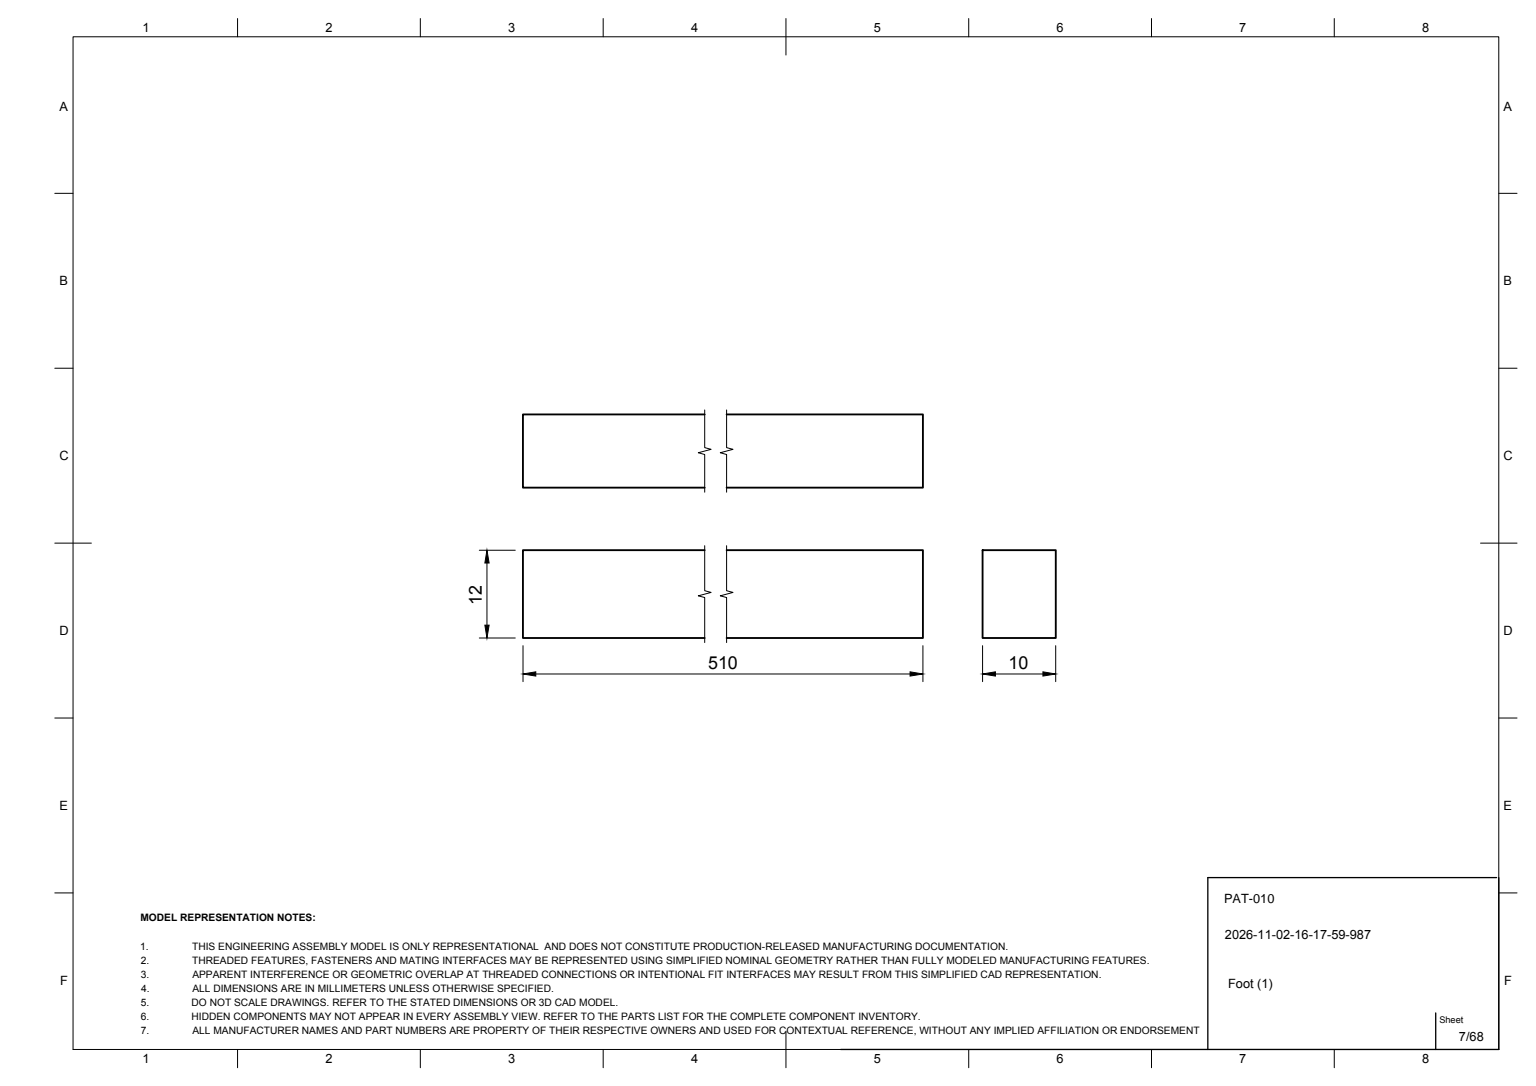
ISO-10303-21;
HEADER;
/* Generated by software containing ST-Developer
 * from STEP Tools, Inc. (www.steptools.com) 
 */

FILE_DESCRIPTION(
/* description */ ('Belt conveyor head drive unit'),
/* implementation_level */ '2;1');

FILE_NAME(
/* name */ 'Foot (1).step',
/* time_stamp */ '2026-10-28T03:26:19-07:00',
/* author */ (''),
/* organization */ (''),
/* preprocessor_version */ 'ST-DEVELOPER v20.2',
/* originating_system */ 'Autodesk Translation Framework v15.17.0.0',
/* authorisation */ '');

FILE_SCHEMA (('AUTOMOTIVE_DESIGN { 1 0 10303 214 3 1 1 }'));
ENDSEC;

DATA;
#10=MECHANICAL_DESIGN_GEOMETRIC_PRESENTATION_REPRESENTATION('',(#849),#27069);
#711=SHAPE_REPRESENTATION_RELATIONSHIP('SRR','None',#27355,#780);
#780=ADVANCED_BREP_SHAPE_REPRESENTATION('',(#934),#26997);
#849=STYLED_ITEM('',(#27811),#934);
#934=MANIFOLD_SOLID_BREP('Body1',#13714);
#1311=PLANE('',#14671);
#1312=PLANE('',#14672);
#1313=PLANE('',#14673);
#1314=PLANE('',#14674);
#1315=PLANE('',#14675);
#1316=PLANE('',#14676);
#1689=FACE_OUTER_BOUND('',#2509,.T.);
#1690=FACE_OUTER_BOUND('',#2510,.T.);
#1691=FACE_OUTER_BOUND('',#2511,.T.);
#1692=FACE_OUTER_BOUND('',#2512,.T.);
#1693=FACE_OUTER_BOUND('',#2513,.T.);
#1694=FACE_OUTER_BOUND('',#2514,.T.);
#2509=EDGE_LOOP('',(#9198,#9199,#9200,#9201));
#2510=EDGE_LOOP('',(#9202,#9203,#9204,#9205));
#2511=EDGE_LOOP('',(#9206,#9207,#9208,#9209));
#2512=EDGE_LOOP('',(#9210,#9211,#9212,#9213));
#2513=EDGE_LOOP('',(#9214,#9215,#9216,#9217));
#2514=EDGE_LOOP('',(#9218,#9219,#9220,#9221));
#3570=LINE('',#21234,#4362);
#3571=LINE('',#21236,#4363);
#3572=LINE('',#21238,#4364);
#3573=LINE('',#21239,#4365);
#3574=LINE('',#21242,#4366);
#3575=LINE('',#21244,#4367);
#3576=LINE('',#21245,#4368);
#3577=LINE('',#21248,#4369);
#3578=LINE('',#21250,#4370);
#3579=LINE('',#21251,#4371);
#3580=LINE('',#21253,#4372);
#3581=LINE('',#21254,#4373);
#4362=VECTOR('',#16726,1.);
#4363=VECTOR('',#16727,1.);
#4364=VECTOR('',#16728,1.);
#4365=VECTOR('',#16729,1.);
#4366=VECTOR('',#16732,1.);
#4367=VECTOR('',#16733,1.);
#4368=VECTOR('',#16734,1.);
#4369=VECTOR('',#16737,1.);
#4370=VECTOR('',#16738,1.);
#4371=VECTOR('',#16739,1.);
#4372=VECTOR('',#16742,1.);
#4373=VECTOR('',#16743,1.);
#6033=VERTEX_POINT('',#21232);
#6034=VERTEX_POINT('',#21233);
#6035=VERTEX_POINT('',#21235);
#6036=VERTEX_POINT('',#21237);
#6037=VERTEX_POINT('',#21241);
#6038=VERTEX_POINT('',#21243);
#6039=VERTEX_POINT('',#21247);
#6040=VERTEX_POINT('',#21249);
#7291=EDGE_CURVE('',#6033,#6034,#3570,.T.);
#7292=EDGE_CURVE('',#6034,#6035,#3571,.T.);
#7293=EDGE_CURVE('',#6036,#6035,#3572,.T.);
#7294=EDGE_CURVE('',#6033,#6036,#3573,.T.);
#7295=EDGE_CURVE('',#6037,#6033,#3574,.T.);
#7296=EDGE_CURVE('',#6038,#6036,#3575,.T.);
#7297=EDGE_CURVE('',#6037,#6038,#3576,.T.);
#7298=EDGE_CURVE('',#6039,#6037,#3577,.T.);
#7299=EDGE_CURVE('',#6040,#6038,#3578,.T.);
#7300=EDGE_CURVE('',#6039,#6040,#3579,.T.);
#7301=EDGE_CURVE('',#6034,#6039,#3580,.T.);
#7302=EDGE_CURVE('',#6035,#6040,#3581,.T.);
#9198=ORIENTED_EDGE('',*,*,#7291,.T.);
#9199=ORIENTED_EDGE('',*,*,#7292,.T.);
#9200=ORIENTED_EDGE('',*,*,#7293,.F.);
#9201=ORIENTED_EDGE('',*,*,#7294,.F.);
#9202=ORIENTED_EDGE('',*,*,#7295,.T.);
#9203=ORIENTED_EDGE('',*,*,#7294,.T.);
#9204=ORIENTED_EDGE('',*,*,#7296,.F.);
#9205=ORIENTED_EDGE('',*,*,#7297,.F.);
#9206=ORIENTED_EDGE('',*,*,#7298,.T.);
#9207=ORIENTED_EDGE('',*,*,#7297,.T.);
#9208=ORIENTED_EDGE('',*,*,#7299,.F.);
#9209=ORIENTED_EDGE('',*,*,#7300,.F.);
#9210=ORIENTED_EDGE('',*,*,#7301,.T.);
#9211=ORIENTED_EDGE('',*,*,#7300,.T.);
#9212=ORIENTED_EDGE('',*,*,#7302,.F.);
#9213=ORIENTED_EDGE('',*,*,#7292,.F.);
#9214=ORIENTED_EDGE('',*,*,#7302,.T.);
#9215=ORIENTED_EDGE('',*,*,#7299,.T.);
#9216=ORIENTED_EDGE('',*,*,#7296,.T.);
#9217=ORIENTED_EDGE('',*,*,#7293,.T.);
#9218=ORIENTED_EDGE('',*,*,#7301,.F.);
#9219=ORIENTED_EDGE('',*,*,#7291,.F.);
#9220=ORIENTED_EDGE('',*,*,#7295,.F.);
#9221=ORIENTED_EDGE('',*,*,#7298,.F.);
#12968=ADVANCED_FACE('',(#1689),#1311,.T.);
#12969=ADVANCED_FACE('',(#1690),#1312,.T.);
#12970=ADVANCED_FACE('',(#1691),#1313,.T.);
#12971=ADVANCED_FACE('',(#1692),#1314,.T.);
#12972=ADVANCED_FACE('',(#1693),#1315,.T.);
#12973=ADVANCED_FACE('',(#1694),#1316,.F.);
#13714=CLOSED_SHELL('',(#12968,#12969,#12970,#12971,#12972,#12973));
#14670=AXIS2_PLACEMENT_3D('',#21230,#16722,#16723);
#14671=AXIS2_PLACEMENT_3D('',#21231,#16724,#16725);
#14672=AXIS2_PLACEMENT_3D('',#21240,#16730,#16731);
#14673=AXIS2_PLACEMENT_3D('',#21246,#16735,#16736);
#14674=AXIS2_PLACEMENT_3D('',#21252,#16740,#16741);
#14675=AXIS2_PLACEMENT_3D('',#21255,#16744,#16745);
#14676=AXIS2_PLACEMENT_3D('',#21256,#16746,#16747);
#16722=DIRECTION('axis',(0.,0.,1.));
#16723=DIRECTION('refdir',(1.,0.,0.));
#16724=DIRECTION('center_axis',(0.,1.,0.));
#16725=DIRECTION('ref_axis',(-1.,0.,0.));
#16726=DIRECTION('',(-1.,0.,0.));
#16727=DIRECTION('',(0.,0.,1.));
#16728=DIRECTION('',(-1.,0.,0.));
#16729=DIRECTION('',(0.,0.,1.));
#16730=DIRECTION('center_axis',(1.,0.,0.));
#16731=DIRECTION('ref_axis',(0.,1.,0.));
#16732=DIRECTION('',(0.,1.,0.));
#16733=DIRECTION('',(0.,1.,0.));
#16734=DIRECTION('',(0.,0.,1.));
#16735=DIRECTION('center_axis',(0.,-1.,0.));
#16736=DIRECTION('ref_axis',(1.,0.,0.));
#16737=DIRECTION('',(1.,0.,0.));
#16738=DIRECTION('',(1.,0.,0.));
#16739=DIRECTION('',(0.,0.,1.));
#16740=DIRECTION('center_axis',(-1.,0.,0.));
#16741=DIRECTION('ref_axis',(0.,-1.,0.));
#16742=DIRECTION('',(0.,-1.,0.));
#16743=DIRECTION('',(0.,-1.,0.));
#16744=DIRECTION('center_axis',(0.,0.,1.));
#16745=DIRECTION('ref_axis',(1.,0.,0.));
#16746=DIRECTION('center_axis',(0.,0.,1.));
#16747=DIRECTION('ref_axis',(1.,0.,0.));
#21230=CARTESIAN_POINT('',(0.,0.,0.));
#21231=CARTESIAN_POINT('Origin',(12.,44.5,-2.4));
#21232=CARTESIAN_POINT('',(12.,44.5,-2.4));
#21233=CARTESIAN_POINT('',(11.,44.5,-2.4));
#21234=CARTESIAN_POINT('',(12.,44.5,-2.4));
#21235=CARTESIAN_POINT('',(11.,44.5,-1.2));
#21236=CARTESIAN_POINT('',(11.,44.5,-2.4));
#21237=CARTESIAN_POINT('',(12.,44.5,-1.2));
#21238=CARTESIAN_POINT('',(12.,44.5,-1.2));
#21239=CARTESIAN_POINT('',(12.,44.5,-2.4));
#21240=CARTESIAN_POINT('Origin',(12.,-6.5,-2.4));
#21241=CARTESIAN_POINT('',(12.,-6.5,-2.4));
#21242=CARTESIAN_POINT('',(12.,-6.5,-2.4));
#21243=CARTESIAN_POINT('',(12.,-6.5,-1.2));
#21244=CARTESIAN_POINT('',(12.,-6.5,-1.2));
#21245=CARTESIAN_POINT('',(12.,-6.5,-2.4));
#21246=CARTESIAN_POINT('Origin',(11.,-6.5,-2.4));
#21247=CARTESIAN_POINT('',(11.,-6.5,-2.4));
#21248=CARTESIAN_POINT('',(11.,-6.5,-2.4));
#21249=CARTESIAN_POINT('',(11.,-6.5,-1.2));
#21250=CARTESIAN_POINT('',(11.,-6.5,-1.2));
#21251=CARTESIAN_POINT('',(11.,-6.5,-2.4));
#21252=CARTESIAN_POINT('Origin',(11.,44.5,-2.4));
#21253=CARTESIAN_POINT('',(11.,44.5,-2.4));
#21254=CARTESIAN_POINT('',(11.,44.5,-1.2));
#21255=CARTESIAN_POINT('Origin',(11.5,19.,-1.2));
#21256=CARTESIAN_POINT('Origin',(11.5,19.,-2.4));
#26920=UNCERTAINTY_MEASURE_WITH_UNIT(LENGTH_MEASURE(0.001),#27070,
'DISTANCE_ACCURACY_VALUE',
'Maximum model space distance between geometric entities at asserted c
onnectivities');
#26992=UNCERTAINTY_MEASURE_WITH_UNIT(LENGTH_MEASURE(0.001),#27070,
'DISTANCE_ACCURACY_VALUE',
'Maximum model space distance between geometric entities at asserted c
onnectivities');
#26997=(
GEOMETRIC_REPRESENTATION_CONTEXT(3)
GLOBAL_UNCERTAINTY_ASSIGNED_CONTEXT((#26920))
GLOBAL_UNIT_ASSIGNED_CONTEXT((#27070,#27072,#27073))
REPRESENTATION_CONTEXT('','3D')
);
#27069=(
GEOMETRIC_REPRESENTATION_CONTEXT(3)
GLOBAL_UNCERTAINTY_ASSIGNED_CONTEXT((#26992))
GLOBAL_UNIT_ASSIGNED_CONTEXT((#27070,#27072,#27073))
REPRESENTATION_CONTEXT('','3D')
);
#27070=(
LENGTH_UNIT()
NAMED_UNIT(*)
SI_UNIT(.CENTI.,.METRE.)
);
#27072=(
NAMED_UNIT(*)
PLANE_ANGLE_UNIT()
SI_UNIT($,.RADIAN.)
);
#27073=(
NAMED_UNIT(*)
SI_UNIT($,.STERADIAN.)
SOLID_ANGLE_UNIT()
);
#27078=SHAPE_DEFINITION_REPRESENTATION(#27154,#27355);
#27154=PRODUCT_DEFINITION_SHAPE('',$,#27432);
#27355=SHAPE_REPRESENTATION('',(#14670),#26997);
#27427=PRODUCT_DEFINITION_CONTEXT('part definition',#27657,'design');
#27432=PRODUCT_DEFINITION('Foot (1)','Foot (1)',#27508,#27427);
#27508=PRODUCT_DEFINITION_FORMATION('',$,#27663);
#27657=APPLICATION_CONTEXT(
'Core Data for Automotive Mechanical Design Process');
#27658=PRODUCT_CONTEXT('part definition',#27657,'mechanical');
#27663=PRODUCT('Foot (1)','Foot (1)','Foot (1)',(#27658));
#27805=COLOUR_RGB('Off White',0.89,0.88,0.83);
#27806=FILL_AREA_STYLE_COLOUR('',#27805);
#27807=FILL_AREA_STYLE('',(#27806));
#27808=SURFACE_STYLE_FILL_AREA(#27807);
#27809=SURFACE_SIDE_STYLE('',(#27808));
#27810=SURFACE_STYLE_USAGE(.BOTH.,#27809);
#27811=PRESENTATION_STYLE_ASSIGNMENT((#27810));
ENDSEC;
END-ISO-10303-21;
